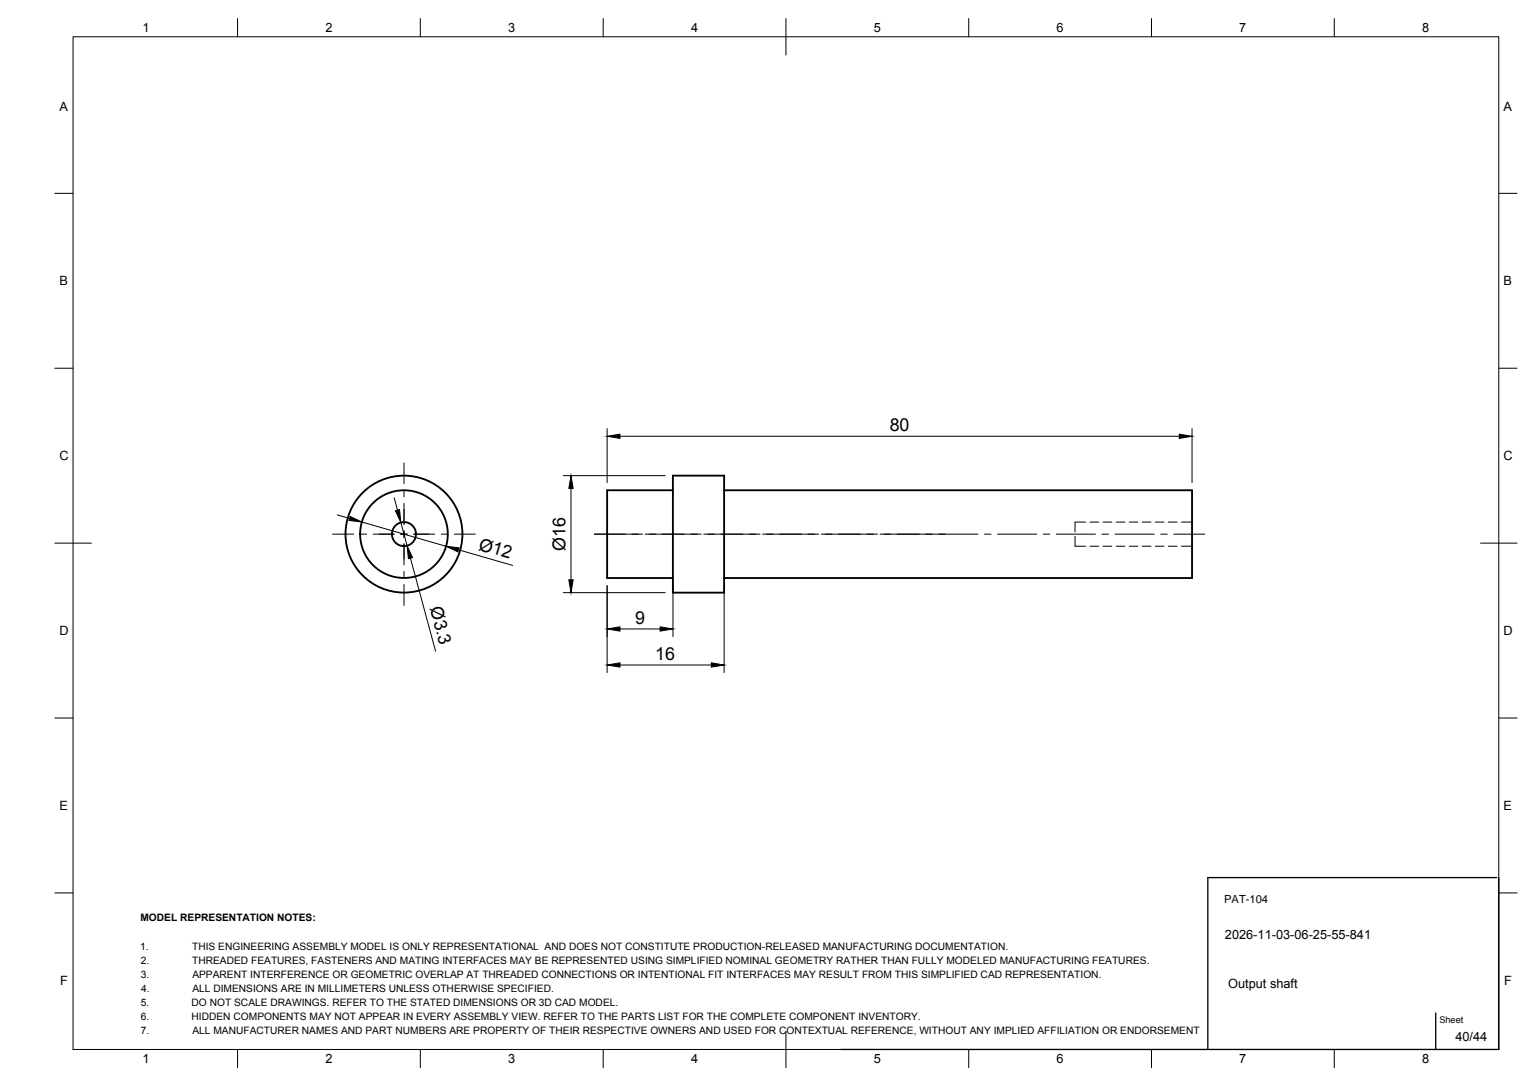
ISO-10303-21;
HEADER;
/* Generated by software containing ST-Developer
 * from STEP Tools, Inc. (www.steptools.com) 
 */

FILE_DESCRIPTION(
/* description */ ('Timing belt drive module 2 mm Pitch Timing 20T-40T'),

/* implementation_level */ '2;1');

FILE_NAME(
/* name */ 'Output shaft.step',
/* time_stamp */ '2026-10-28T03:25:12-07:00',
/* author */ (''),
/* organization */ (''),
/* preprocessor_version */ 'ST-DEVELOPER v20.2',
/* originating_system */ 'Autodesk Translation Framework v15.17.0.0',
/* authorisation */ '');

FILE_SCHEMA (('AUTOMOTIVE_DESIGN { 1 0 10303 214 3 1 1 }'));
ENDSEC;

DATA;
#10=MECHANICAL_DESIGN_GEOMETRIC_PRESENTATION_REPRESENTATION('',(#574),#17830);
#473=SHAPE_REPRESENTATION_RELATIONSHIP('SRR','None',#18047,#516);
#516=ADVANCED_BREP_SHAPE_REPRESENTATION('',(#630),#17822);
#574=STYLED_ITEM('',(#18317),#630);
#630=MANIFOLD_SOLID_BREP('Body1',#9033);
#752=FACE_BOUND('',#1985,.T.);
#753=FACE_BOUND('',#1987,.T.);
#754=FACE_BOUND('',#1991,.T.);
#931=PLANE('',#10405);
#932=PLANE('',#10406);
#933=PLANE('',#10409);
#934=PLANE('',#10415);
#935=PLANE('',#10418);
#1346=FACE_OUTER_BOUND('',#1982,.T.);
#1347=FACE_OUTER_BOUND('',#1983,.T.);
#1348=FACE_OUTER_BOUND('',#1984,.T.);
#1349=FACE_OUTER_BOUND('',#1986,.T.);
#1350=FACE_OUTER_BOUND('',#1988,.T.);
#1351=FACE_OUTER_BOUND('',#1989,.T.);
#1352=FACE_OUTER_BOUND('',#1990,.T.);
#1353=FACE_OUTER_BOUND('',#1992,.T.);
#1354=FACE_OUTER_BOUND('',#1993,.T.);
#1982=EDGE_LOOP('',(#7485,#7486,#7487,#7488));
#1983=EDGE_LOOP('',(#7489));
#1984=EDGE_LOOP('',(#7490));
#1985=EDGE_LOOP('',(#7491));
#1986=EDGE_LOOP('',(#7492));
#1987=EDGE_LOOP('',(#7493));
#1988=EDGE_LOOP('',(#7494,#7495,#7496,#7497));
#1989=EDGE_LOOP('',(#7498,#7499,#7500,#7501));
#1990=EDGE_LOOP('',(#7502));
#1991=EDGE_LOOP('',(#7503));
#1992=EDGE_LOOP('',(#7504,#7505,#7506,#7507));
#1993=EDGE_LOOP('',(#7508));
#2590=CIRCLE('',#10403,0.165);
#2591=CIRCLE('',#10404,0.165);
#2592=CIRCLE('',#10407,0.8);
#2593=CIRCLE('',#10408,0.6);
#2594=CIRCLE('',#10410,0.8);
#2595=CIRCLE('',#10411,0.6);
#2596=CIRCLE('',#10414,0.6);
#2597=CIRCLE('',#10417,0.6);
#3142=LINE('',#16668,#3620);
#3143=LINE('',#16682,#3621);
#3144=LINE('',#16685,#3622);
#3145=LINE('',#16691,#3623);
#3620=VECTOR('',#12937,0.165);
#3621=VECTOR('',#12956,0.8);
#3622=VECTOR('',#12959,0.6);
#3623=VECTOR('',#12968,0.6);
#4335=VERTEX_POINT('',#16665);
#4336=VERTEX_POINT('',#16667);
#4337=VERTEX_POINT('',#16672);
#4338=VERTEX_POINT('',#16674);
#4339=VERTEX_POINT('',#16677);
#4340=VERTEX_POINT('',#16679);
#4341=VERTEX_POINT('',#16684);
#4342=VERTEX_POINT('',#16689);
#5425=EDGE_CURVE('',#4335,#4335,#2590,.T.);
#5426=EDGE_CURVE('',#4335,#4336,#3142,.T.);
#5427=EDGE_CURVE('',#4336,#4336,#2591,.T.);
#5428=EDGE_CURVE('',#4337,#4337,#2592,.T.);
#5429=EDGE_CURVE('',#4338,#4338,#2593,.T.);
#5430=EDGE_CURVE('',#4339,#4339,#2594,.T.);
#5431=EDGE_CURVE('',#4340,#4340,#2595,.T.);
#5432=EDGE_CURVE('',#4337,#4339,#3143,.T.);
#5433=EDGE_CURVE('',#4340,#4341,#3144,.T.);
#5434=EDGE_CURVE('',#4341,#4341,#2596,.T.);
#5435=EDGE_CURVE('',#4342,#4342,#2597,.T.);
#5436=EDGE_CURVE('',#4342,#4338,#3145,.T.);
#7485=ORIENTED_EDGE('',*,*,#5425,.F.);
#7486=ORIENTED_EDGE('',*,*,#5426,.T.);
#7487=ORIENTED_EDGE('',*,*,#5427,.T.);
#7488=ORIENTED_EDGE('',*,*,#5426,.F.);
#7489=ORIENTED_EDGE('',*,*,#5427,.F.);
#7490=ORIENTED_EDGE('',*,*,#5428,.T.);
#7491=ORIENTED_EDGE('',*,*,#5429,.F.);
#7492=ORIENTED_EDGE('',*,*,#5430,.F.);
#7493=ORIENTED_EDGE('',*,*,#5431,.F.);
#7494=ORIENTED_EDGE('',*,*,#5428,.F.);
#7495=ORIENTED_EDGE('',*,*,#5432,.T.);
#7496=ORIENTED_EDGE('',*,*,#5430,.T.);
#7497=ORIENTED_EDGE('',*,*,#5432,.F.);
#7498=ORIENTED_EDGE('',*,*,#5431,.T.);
#7499=ORIENTED_EDGE('',*,*,#5433,.T.);
#7500=ORIENTED_EDGE('',*,*,#5434,.T.);
#7501=ORIENTED_EDGE('',*,*,#5433,.F.);
#7502=ORIENTED_EDGE('',*,*,#5434,.F.);
#7503=ORIENTED_EDGE('',*,*,#5425,.T.);
#7504=ORIENTED_EDGE('',*,*,#5435,.F.);
#7505=ORIENTED_EDGE('',*,*,#5436,.T.);
#7506=ORIENTED_EDGE('',*,*,#5429,.T.);
#7507=ORIENTED_EDGE('',*,*,#5436,.F.);
#7508=ORIENTED_EDGE('',*,*,#5435,.T.);
#8358=CYLINDRICAL_SURFACE('',#10402,0.165);
#8359=CYLINDRICAL_SURFACE('',#10412,0.8);
#8360=CYLINDRICAL_SURFACE('',#10413,0.6);
#8361=CYLINDRICAL_SURFACE('',#10416,0.6);
#8844=ADVANCED_FACE('',(#1346),#8358,.F.);
#8845=ADVANCED_FACE('',(#1347),#931,.F.);
#8846=ADVANCED_FACE('',(#1348,#752),#932,.T.);
#8847=ADVANCED_FACE('',(#1349,#753),#933,.F.);
#8848=ADVANCED_FACE('',(#1350),#8359,.T.);
#8849=ADVANCED_FACE('',(#1351),#8360,.T.);
#8850=ADVANCED_FACE('',(#1352,#754),#934,.F.);
#8851=ADVANCED_FACE('',(#1353),#8361,.T.);
#8852=ADVANCED_FACE('',(#1354),#935,.T.);
#9033=CLOSED_SHELL('',(#8844,#8845,#8846,#8847,#8848,#8849,#8850,#8851,
#8852));
#10401=AXIS2_PLACEMENT_3D('',#16663,#12931,#12932);
#10402=AXIS2_PLACEMENT_3D('',#16664,#12933,#12934);
#10403=AXIS2_PLACEMENT_3D('',#16666,#12935,#12936);
#10404=AXIS2_PLACEMENT_3D('',#16669,#12938,#12939);
#10405=AXIS2_PLACEMENT_3D('',#16670,#12940,#12941);
#10406=AXIS2_PLACEMENT_3D('',#16671,#12942,#12943);
#10407=AXIS2_PLACEMENT_3D('',#16673,#12944,#12945);
#10408=AXIS2_PLACEMENT_3D('',#16675,#12946,#12947);
#10409=AXIS2_PLACEMENT_3D('',#16676,#12948,#12949);
#10410=AXIS2_PLACEMENT_3D('',#16678,#12950,#12951);
#10411=AXIS2_PLACEMENT_3D('',#16680,#12952,#12953);
#10412=AXIS2_PLACEMENT_3D('',#16681,#12954,#12955);
#10413=AXIS2_PLACEMENT_3D('',#16683,#12957,#12958);
#10414=AXIS2_PLACEMENT_3D('',#16686,#12960,#12961);
#10415=AXIS2_PLACEMENT_3D('',#16687,#12962,#12963);
#10416=AXIS2_PLACEMENT_3D('',#16688,#12964,#12965);
#10417=AXIS2_PLACEMENT_3D('',#16690,#12966,#12967);
#10418=AXIS2_PLACEMENT_3D('',#16692,#12969,#12970);
#12931=DIRECTION('axis',(0.,0.,1.));
#12932=DIRECTION('refdir',(1.,0.,0.));
#12933=DIRECTION('center_axis',(0.,1.,0.));
#12934=DIRECTION('ref_axis',(1.,0.,0.));
#12935=DIRECTION('center_axis',(0.,1.,0.));
#12936=DIRECTION('ref_axis',(1.,0.,0.));
#12937=DIRECTION('',(0.,1.,0.));
#12938=DIRECTION('center_axis',(0.,1.,0.));
#12939=DIRECTION('ref_axis',(1.,0.,0.));
#12940=DIRECTION('center_axis',(0.,1.,0.));
#12941=DIRECTION('ref_axis',(1.,0.,0.));
#12942=DIRECTION('center_axis',(0.,1.,0.));
#12943=DIRECTION('ref_axis',(1.,0.,0.));
#12944=DIRECTION('center_axis',(0.,1.,0.));
#12945=DIRECTION('ref_axis',(1.,0.,0.));
#12946=DIRECTION('center_axis',(0.,1.,0.));
#12947=DIRECTION('ref_axis',(1.,0.,0.));
#12948=DIRECTION('center_axis',(0.,1.,0.));
#12949=DIRECTION('ref_axis',(1.,0.,0.));
#12950=DIRECTION('center_axis',(0.,1.,0.));
#12951=DIRECTION('ref_axis',(1.,0.,0.));
#12952=DIRECTION('center_axis',(0.,-1.,0.));
#12953=DIRECTION('ref_axis',(1.,0.,0.));
#12954=DIRECTION('center_axis',(0.,1.,0.));
#12955=DIRECTION('ref_axis',(1.,0.,0.));
#12956=DIRECTION('',(0.,-1.,0.));
#12957=DIRECTION('center_axis',(0.,1.,0.));
#12958=DIRECTION('ref_axis',(1.,0.,0.));
#12959=DIRECTION('',(0.,-1.,0.));
#12960=DIRECTION('center_axis',(0.,1.,0.));
#12961=DIRECTION('ref_axis',(1.,0.,0.));
#12962=DIRECTION('center_axis',(0.,1.,0.));
#12963=DIRECTION('ref_axis',(1.,0.,0.));
#12964=DIRECTION('center_axis',(0.,1.,0.));
#12965=DIRECTION('ref_axis',(1.,0.,0.));
#12966=DIRECTION('center_axis',(0.,1.,0.));
#12967=DIRECTION('ref_axis',(1.,0.,0.));
#12968=DIRECTION('',(0.,-1.,0.));
#12969=DIRECTION('center_axis',(0.,1.,0.));
#12970=DIRECTION('ref_axis',(1.,0.,0.));
#16663=CARTESIAN_POINT('',(0.,0.,0.));
#16664=CARTESIAN_POINT('Origin',(6.97091003018116,-5.1,7.));
#16665=CARTESIAN_POINT('',(6.80591003018116,-5.,7.));
#16666=CARTESIAN_POINT('Origin',(6.97091003018116,-5.,7.));
#16667=CARTESIAN_POINT('',(6.80591003018116,-3.4,7.));
#16668=CARTESIAN_POINT('',(6.80591003018116,-5.1,7.));
#16669=CARTESIAN_POINT('Origin',(6.97091003018116,-3.4,7.));
#16670=CARTESIAN_POINT('Origin',(6.97091003018116,-3.4,7.));
#16671=CARTESIAN_POINT('Origin',(6.97091003018116,2.1,7.));
#16672=CARTESIAN_POINT('',(6.17091003018116,2.1,7.));
#16673=CARTESIAN_POINT('Origin',(6.97091003018116,2.1,7.));
#16674=CARTESIAN_POINT('',(6.37091003018116,2.1,7.));
#16675=CARTESIAN_POINT('Origin',(6.97091003018116,2.1,7.));
#16676=CARTESIAN_POINT('Origin',(6.97091003018116,1.4,7.));
#16677=CARTESIAN_POINT('',(6.17091003018116,1.4,7.));
#16678=CARTESIAN_POINT('Origin',(6.97091003018116,1.4,7.));
#16679=CARTESIAN_POINT('',(6.37091003018116,1.4,7.));
#16680=CARTESIAN_POINT('Origin',(6.97091003018116,1.4,7.));
#16681=CARTESIAN_POINT('Origin',(6.97091003018116,1.4,7.));
#16682=CARTESIAN_POINT('',(6.17091003018116,1.4,7.));
#16683=CARTESIAN_POINT('Origin',(6.97091003018116,-1.8,7.));
#16684=CARTESIAN_POINT('',(6.37091003018116,-5.,7.));
#16685=CARTESIAN_POINT('',(6.37091003018116,-1.8,7.));
#16686=CARTESIAN_POINT('Origin',(6.97091003018116,-5.,7.));
#16687=CARTESIAN_POINT('Origin',(6.97091003018116,-5.,7.));
#16688=CARTESIAN_POINT('Origin',(6.97091003018116,-1.8,7.));
#16689=CARTESIAN_POINT('',(6.37091003018116,3.,7.));
#16690=CARTESIAN_POINT('Origin',(6.97091003018116,3.,7.));
#16691=CARTESIAN_POINT('',(6.37091003018116,-1.8,7.));
#16692=CARTESIAN_POINT('Origin',(6.97091003018116,3.,7.));
#17772=UNCERTAINTY_MEASURE_WITH_UNIT(LENGTH_MEASURE(0.001),#17831,
'DISTANCE_ACCURACY_VALUE',
'Maximum model space distance between geometric entities at asserted c
onnectivities');
#17780=UNCERTAINTY_MEASURE_WITH_UNIT(LENGTH_MEASURE(0.001),#17831,
'DISTANCE_ACCURACY_VALUE',
'Maximum model space distance between geometric entities at asserted c
onnectivities');
#17822=(
GEOMETRIC_REPRESENTATION_CONTEXT(3)
GLOBAL_UNCERTAINTY_ASSIGNED_CONTEXT((#17772))
GLOBAL_UNIT_ASSIGNED_CONTEXT((#17831,#17833,#17834))
REPRESENTATION_CONTEXT('','3D')
);
#17830=(
GEOMETRIC_REPRESENTATION_CONTEXT(3)
GLOBAL_UNCERTAINTY_ASSIGNED_CONTEXT((#17780))
GLOBAL_UNIT_ASSIGNED_CONTEXT((#17831,#17833,#17834))
REPRESENTATION_CONTEXT('','3D')
);
#17831=(
LENGTH_UNIT()
NAMED_UNIT(*)
SI_UNIT(.CENTI.,.METRE.)
);
#17833=(
NAMED_UNIT(*)
PLANE_ANGLE_UNIT()
SI_UNIT($,.RADIAN.)
);
#17834=(
NAMED_UNIT(*)
SI_UNIT($,.STERADIAN.)
SOLID_ANGLE_UNIT()
);
#17876=SHAPE_DEFINITION_REPRESENTATION(#17935,#18047);
#17935=PRODUCT_DEFINITION_SHAPE('',$,#18097);
#18047=SHAPE_REPRESENTATION('',(#10401),#17822);
#18055=PRODUCT_DEFINITION_CONTEXT('part definition',#18204,'design');
#18097=PRODUCT_DEFINITION('Output shaft','Output shaft',#18146,#18055);
#18146=PRODUCT_DEFINITION_FORMATION('',$,#18247);
#18204=APPLICATION_CONTEXT(
'Core Data for Automotive Mechanical Design Process');
#18205=PRODUCT_CONTEXT('part definition',#18204,'mechanical');
#18247=PRODUCT('Output shaft','Output shaft','Output shaft',(#18205));
#18311=COLOUR_RGB('Grey',0.48,0.52,0.57);
#18312=FILL_AREA_STYLE_COLOUR('',#18311);
#18313=FILL_AREA_STYLE('',(#18312));
#18314=SURFACE_STYLE_FILL_AREA(#18313);
#18315=SURFACE_SIDE_STYLE('',(#18314));
#18316=SURFACE_STYLE_USAGE(.BOTH.,#18315);
#18317=PRESENTATION_STYLE_ASSIGNMENT((#18316));
ENDSEC;
END-ISO-10303-21;
